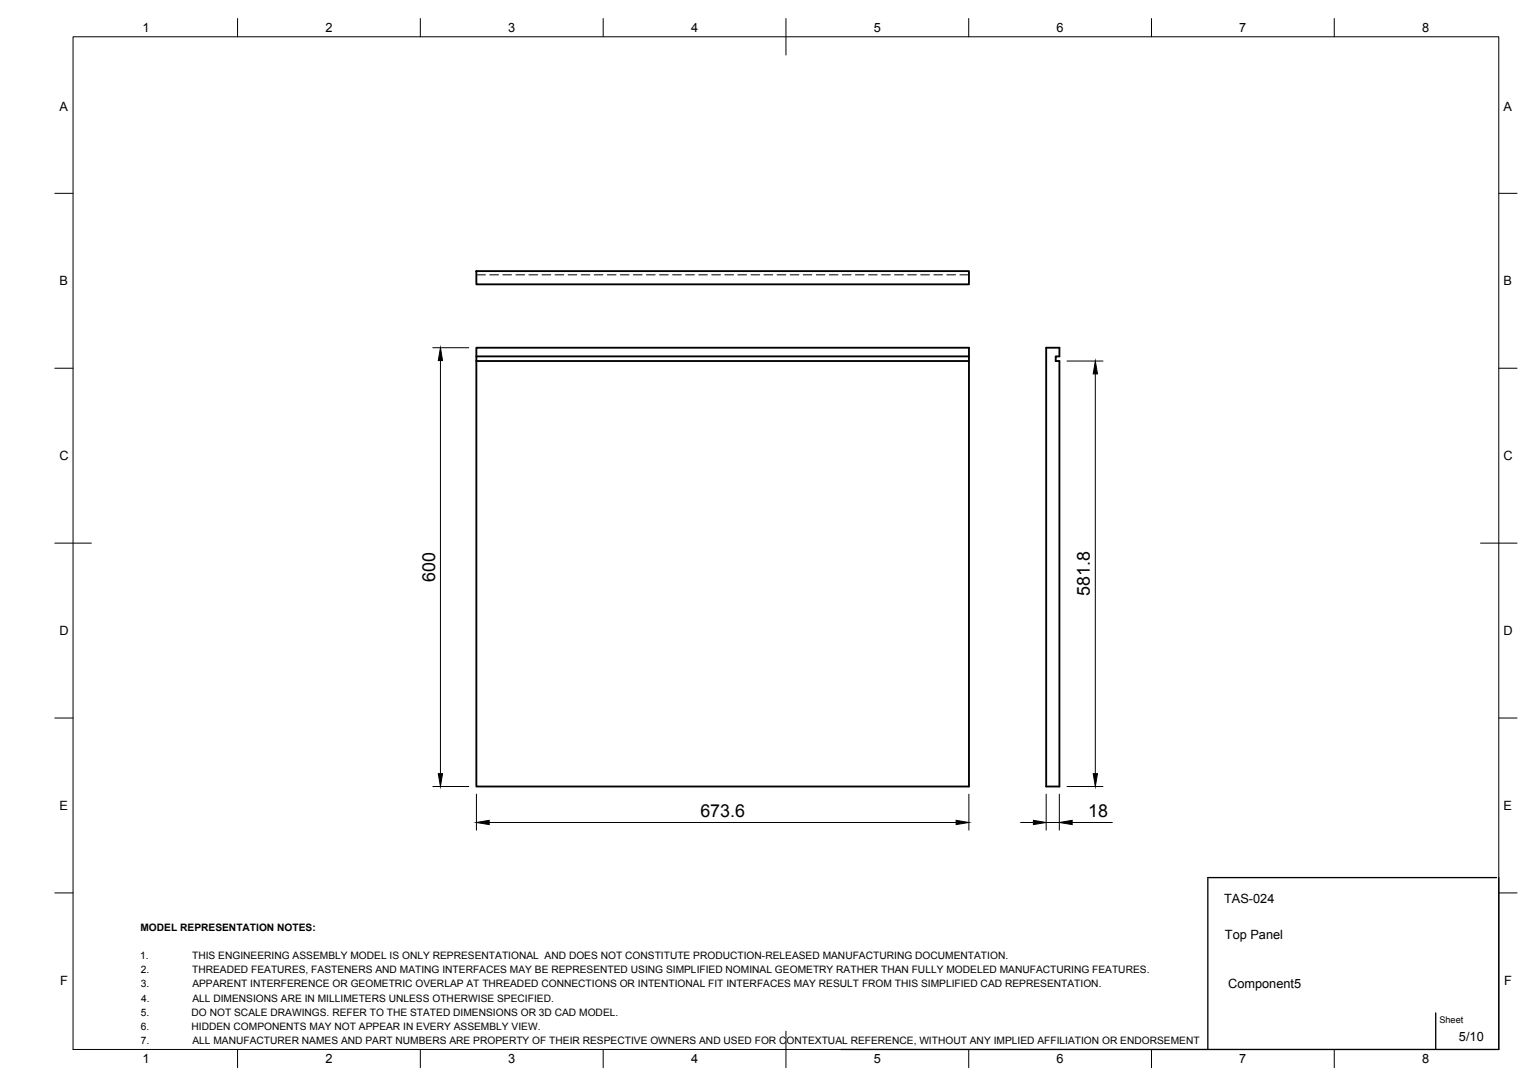
ISO-10303-21;
HEADER;
/* Generated by software containing ST-Developer
 * from STEP Tools, Inc. (www.steptools.com) 
 */

FILE_DESCRIPTION(
/* description */ (''),
/* implementation_level */ '2;1');

FILE_NAME(
/* name */ 'Top panel.step',
/* time_stamp */ '2026-11-15T17:53:25-08:00',
/* author */ (''),
/* organization */ (''),
/* preprocessor_version */ 'ST-DEVELOPER v20.2',
/* originating_system */ 'Autodesk Translation Framework v15.17.0.0',
/* authorisation */ '');

FILE_SCHEMA (('AUTOMOTIVE_DESIGN { 1 0 10303 214 3 1 1 }'));
ENDSEC;

DATA;
#10=MECHANICAL_DESIGN_GEOMETRIC_PRESENTATION_REPRESENTATION('',(#133),#2673);
#117=SHAPE_REPRESENTATION_RELATIONSHIP('SRR','None',#2725,#125);
#125=ADVANCED_BREP_SHAPE_REPRESENTATION('',(#141),#2667);
#133=STYLED_ITEM('',(#2774),#141);
#141=MANIFOLD_SOLID_BREP('Body1',#1519);
#202=PLANE('',#1690);
#203=PLANE('',#1691);
#204=PLANE('',#1692);
#205=PLANE('',#1693);
#206=PLANE('',#1694);
#207=PLANE('',#1695);
#208=PLANE('',#1696);
#209=PLANE('',#1697);
#210=PLANE('',#1698);
#211=PLANE('',#1699);
#285=FACE_OUTER_BOUND('',#384,.T.);
#286=FACE_OUTER_BOUND('',#385,.T.);
#287=FACE_OUTER_BOUND('',#386,.T.);
#288=FACE_OUTER_BOUND('',#387,.T.);
#289=FACE_OUTER_BOUND('',#388,.T.);
#290=FACE_OUTER_BOUND('',#389,.T.);
#291=FACE_OUTER_BOUND('',#390,.T.);
#292=FACE_OUTER_BOUND('',#391,.T.);
#293=FACE_OUTER_BOUND('',#392,.T.);
#294=FACE_OUTER_BOUND('',#393,.T.);
#384=EDGE_LOOP('',(#1280,#1281,#1282,#1283));
#385=EDGE_LOOP('',(#1284,#1285,#1286,#1287));
#386=EDGE_LOOP('',(#1288,#1289,#1290,#1291));
#387=EDGE_LOOP('',(#1292,#1293,#1294,#1295,#1296,#1297,#1298,#1299));
#388=EDGE_LOOP('',(#1300,#1301,#1302,#1303));
#389=EDGE_LOOP('',(#1304,#1305,#1306,#1307));
#390=EDGE_LOOP('',(#1308,#1309,#1310,#1311));
#391=EDGE_LOOP('',(#1312,#1313,#1314,#1315,#1316,#1317,#1318,#1319));
#392=EDGE_LOOP('',(#1320,#1321,#1322,#1323));
#393=EDGE_LOOP('',(#1324,#1325,#1326,#1327));
#518=LINE('',#2479,#666);
#519=LINE('',#2481,#667);
#520=LINE('',#2483,#668);
#521=LINE('',#2484,#669);
#522=LINE('',#2488,#670);
#523=LINE('',#2490,#671);
#524=LINE('',#2492,#672);
#525=LINE('',#2493,#673);
#526=LINE('',#2495,#674);
#527=LINE('',#2496,#675);
#528=LINE('',#2499,#676);
#529=LINE('',#2501,#677);
#530=LINE('',#2503,#678);
#531=LINE('',#2505,#679);
#532=LINE('',#2506,#680);
#533=LINE('',#2509,#681);
#534=LINE('',#2510,#682);
#535=LINE('',#2513,#683);
#536=LINE('',#2515,#684);
#537=LINE('',#2516,#685);
#538=LINE('',#2519,#686);
#539=LINE('',#2520,#687);
#540=LINE('',#2522,#688);
#541=LINE('',#2523,#689);
#666=VECTOR('',#2018,1.);
#667=VECTOR('',#2019,1.);
#668=VECTOR('',#2020,1.);
#669=VECTOR('',#2021,1.);
#670=VECTOR('',#2024,1.);
#671=VECTOR('',#2025,1.);
#672=VECTOR('',#2026,1.);
#673=VECTOR('',#2027,1.);
#674=VECTOR('',#2030,1.);
#675=VECTOR('',#2031,1.);
#676=VECTOR('',#2034,1.);
#677=VECTOR('',#2035,1.);
#678=VECTOR('',#2036,1.);
#679=VECTOR('',#2037,1.);
#680=VECTOR('',#2038,1.);
#681=VECTOR('',#2041,1.);
#682=VECTOR('',#2042,1.);
#683=VECTOR('',#2045,1.);
#684=VECTOR('',#2046,1.);
#685=VECTOR('',#2047,1.);
#686=VECTOR('',#2050,1.);
#687=VECTOR('',#2051,1.);
#688=VECTOR('',#2054,1.);
#689=VECTOR('',#2055,1.);
#828=VERTEX_POINT('',#2477);
#829=VERTEX_POINT('',#2478);
#830=VERTEX_POINT('',#2480);
#831=VERTEX_POINT('',#2482);
#832=VERTEX_POINT('',#2486);
#833=VERTEX_POINT('',#2487);
#834=VERTEX_POINT('',#2489);
#835=VERTEX_POINT('',#2491);
#836=VERTEX_POINT('',#2498);
#837=VERTEX_POINT('',#2500);
#838=VERTEX_POINT('',#2502);
#839=VERTEX_POINT('',#2504);
#840=VERTEX_POINT('',#2508);
#841=VERTEX_POINT('',#2512);
#842=VERTEX_POINT('',#2514);
#843=VERTEX_POINT('',#2518);
#986=EDGE_CURVE('',#828,#829,#518,.T.);
#987=EDGE_CURVE('',#830,#828,#519,.T.);
#988=EDGE_CURVE('',#831,#830,#520,.T.);
#989=EDGE_CURVE('',#829,#831,#521,.T.);
#990=EDGE_CURVE('',#832,#833,#522,.T.);
#991=EDGE_CURVE('',#834,#832,#523,.T.);
#992=EDGE_CURVE('',#835,#834,#524,.T.);
#993=EDGE_CURVE('',#833,#835,#525,.T.);
#994=EDGE_CURVE('',#831,#834,#526,.T.);
#995=EDGE_CURVE('',#835,#830,#527,.T.);
#996=EDGE_CURVE('',#836,#828,#528,.T.);
#997=EDGE_CURVE('',#837,#836,#529,.T.);
#998=EDGE_CURVE('',#837,#838,#530,.T.);
#999=EDGE_CURVE('',#838,#839,#531,.T.);
#1000=EDGE_CURVE('',#833,#839,#532,.T.);
#1001=EDGE_CURVE('',#829,#840,#533,.T.);
#1002=EDGE_CURVE('',#840,#836,#534,.T.);
#1003=EDGE_CURVE('',#838,#841,#535,.T.);
#1004=EDGE_CURVE('',#841,#842,#536,.T.);
#1005=EDGE_CURVE('',#839,#842,#537,.T.);
#1006=EDGE_CURVE('',#843,#837,#538,.T.);
#1007=EDGE_CURVE('',#843,#840,#539,.T.);
#1008=EDGE_CURVE('',#842,#832,#540,.T.);
#1009=EDGE_CURVE('',#841,#843,#541,.T.);
#1280=ORIENTED_EDGE('',*,*,#986,.F.);
#1281=ORIENTED_EDGE('',*,*,#987,.F.);
#1282=ORIENTED_EDGE('',*,*,#988,.F.);
#1283=ORIENTED_EDGE('',*,*,#989,.F.);
#1284=ORIENTED_EDGE('',*,*,#990,.F.);
#1285=ORIENTED_EDGE('',*,*,#991,.F.);
#1286=ORIENTED_EDGE('',*,*,#992,.F.);
#1287=ORIENTED_EDGE('',*,*,#993,.F.);
#1288=ORIENTED_EDGE('',*,*,#994,.F.);
#1289=ORIENTED_EDGE('',*,*,#988,.T.);
#1290=ORIENTED_EDGE('',*,*,#995,.F.);
#1291=ORIENTED_EDGE('',*,*,#992,.T.);
#1292=ORIENTED_EDGE('',*,*,#993,.T.);
#1293=ORIENTED_EDGE('',*,*,#995,.T.);
#1294=ORIENTED_EDGE('',*,*,#987,.T.);
#1295=ORIENTED_EDGE('',*,*,#996,.F.);
#1296=ORIENTED_EDGE('',*,*,#997,.F.);
#1297=ORIENTED_EDGE('',*,*,#998,.T.);
#1298=ORIENTED_EDGE('',*,*,#999,.T.);
#1299=ORIENTED_EDGE('',*,*,#1000,.F.);
#1300=ORIENTED_EDGE('',*,*,#986,.T.);
#1301=ORIENTED_EDGE('',*,*,#1001,.T.);
#1302=ORIENTED_EDGE('',*,*,#1002,.T.);
#1303=ORIENTED_EDGE('',*,*,#996,.T.);
#1304=ORIENTED_EDGE('',*,*,#1003,.T.);
#1305=ORIENTED_EDGE('',*,*,#1004,.T.);
#1306=ORIENTED_EDGE('',*,*,#1005,.F.);
#1307=ORIENTED_EDGE('',*,*,#999,.F.);
#1308=ORIENTED_EDGE('',*,*,#1006,.T.);
#1309=ORIENTED_EDGE('',*,*,#997,.T.);
#1310=ORIENTED_EDGE('',*,*,#1002,.F.);
#1311=ORIENTED_EDGE('',*,*,#1007,.F.);
#1312=ORIENTED_EDGE('',*,*,#991,.T.);
#1313=ORIENTED_EDGE('',*,*,#1008,.F.);
#1314=ORIENTED_EDGE('',*,*,#1004,.F.);
#1315=ORIENTED_EDGE('',*,*,#1009,.T.);
#1316=ORIENTED_EDGE('',*,*,#1007,.T.);
#1317=ORIENTED_EDGE('',*,*,#1001,.F.);
#1318=ORIENTED_EDGE('',*,*,#989,.T.);
#1319=ORIENTED_EDGE('',*,*,#994,.T.);
#1320=ORIENTED_EDGE('',*,*,#990,.T.);
#1321=ORIENTED_EDGE('',*,*,#1000,.T.);
#1322=ORIENTED_EDGE('',*,*,#1005,.T.);
#1323=ORIENTED_EDGE('',*,*,#1008,.T.);
#1324=ORIENTED_EDGE('',*,*,#1009,.F.);
#1325=ORIENTED_EDGE('',*,*,#1003,.F.);
#1326=ORIENTED_EDGE('',*,*,#998,.F.);
#1327=ORIENTED_EDGE('',*,*,#1006,.F.);
#1480=ADVANCED_FACE('',(#285),#202,.F.);
#1481=ADVANCED_FACE('',(#286),#203,.F.);
#1482=ADVANCED_FACE('',(#287),#204,.T.);
#1483=ADVANCED_FACE('',(#288),#205,.T.);
#1484=ADVANCED_FACE('',(#289),#206,.T.);
#1485=ADVANCED_FACE('',(#290),#207,.T.);
#1486=ADVANCED_FACE('',(#291),#208,.T.);
#1487=ADVANCED_FACE('',(#292),#209,.T.);
#1488=ADVANCED_FACE('',(#293),#210,.T.);
#1489=ADVANCED_FACE('',(#294),#211,.F.);
#1519=CLOSED_SHELL('',(#1480,#1481,#1482,#1483,#1484,#1485,#1486,#1487,
#1488,#1489));
#1689=AXIS2_PLACEMENT_3D('',#2475,#2014,#2015);
#1690=AXIS2_PLACEMENT_3D('',#2476,#2016,#2017);
#1691=AXIS2_PLACEMENT_3D('',#2485,#2022,#2023);
#1692=AXIS2_PLACEMENT_3D('',#2494,#2028,#2029);
#1693=AXIS2_PLACEMENT_3D('',#2497,#2032,#2033);
#1694=AXIS2_PLACEMENT_3D('',#2507,#2039,#2040);
#1695=AXIS2_PLACEMENT_3D('',#2511,#2043,#2044);
#1696=AXIS2_PLACEMENT_3D('',#2517,#2048,#2049);
#1697=AXIS2_PLACEMENT_3D('',#2521,#2052,#2053);
#1698=AXIS2_PLACEMENT_3D('',#2524,#2056,#2057);
#1699=AXIS2_PLACEMENT_3D('',#2525,#2058,#2059);
#2014=DIRECTION('axis',(0.,0.,1.));
#2015=DIRECTION('refdir',(1.,0.,0.));
#2016=DIRECTION('center_axis',(0.,-1.,0.));
#2017=DIRECTION('ref_axis',(1.,0.,0.));
#2018=DIRECTION('',(-1.,0.,0.));
#2019=DIRECTION('',(0.,0.,1.));
#2020=DIRECTION('',(1.,0.,0.));
#2021=DIRECTION('',(0.,0.,-1.));
#2022=DIRECTION('center_axis',(0.,1.,0.));
#2023=DIRECTION('ref_axis',(-1.,0.,0.));
#2024=DIRECTION('',(1.,0.,0.));
#2025=DIRECTION('',(0.,0.,1.));
#2026=DIRECTION('',(-1.,0.,0.));
#2027=DIRECTION('',(0.,0.,-1.));
#2028=DIRECTION('center_axis',(0.,0.,1.));
#2029=DIRECTION('ref_axis',(1.,0.,0.));
#2030=DIRECTION('',(0.,1.,0.));
#2031=DIRECTION('',(0.,-1.,0.));
#2032=DIRECTION('center_axis',(1.,0.,0.));
#2033=DIRECTION('ref_axis',(0.,1.,0.));
#2034=DIRECTION('',(0.,1.,0.));
#2035=DIRECTION('',(0.,0.,1.));
#2036=DIRECTION('',(0.,1.,0.));
#2037=DIRECTION('',(0.,0.,1.));
#2038=DIRECTION('',(0.,1.,0.));
#2039=DIRECTION('center_axis',(0.,0.,1.));
#2040=DIRECTION('ref_axis',(1.,0.,0.));
#2041=DIRECTION('',(0.,-1.,0.));
#2042=DIRECTION('',(1.,0.,0.));
#2043=DIRECTION('center_axis',(0.,1.,0.));
#2044=DIRECTION('ref_axis',(-1.,0.,0.));
#2045=DIRECTION('',(-1.,0.,0.));
#2046=DIRECTION('',(0.,0.,1.));
#2047=DIRECTION('',(-1.,0.,0.));
#2048=DIRECTION('center_axis',(0.,-1.,0.));
#2049=DIRECTION('ref_axis',(1.,0.,0.));
#2050=DIRECTION('',(1.,0.,0.));
#2051=DIRECTION('',(0.,0.,1.));
#2052=DIRECTION('center_axis',(-1.,0.,0.));
#2053=DIRECTION('ref_axis',(0.,-1.,0.));
#2054=DIRECTION('',(0.,-1.,0.));
#2055=DIRECTION('',(0.,-1.,0.));
#2056=DIRECTION('center_axis',(0.,0.,1.));
#2057=DIRECTION('ref_axis',(1.,0.,0.));
#2058=DIRECTION('center_axis',(0.,0.,1.));
#2059=DIRECTION('ref_axis',(1.,0.,0.));
#2475=CARTESIAN_POINT('',(0.,0.,0.));
#2476=CARTESIAN_POINT('Origin',(0.,58.18,1.3));
#2477=CARTESIAN_POINT('',(67.36,58.18,1.8));
#2478=CARTESIAN_POINT('',(0.,58.18,1.8));
#2479=CARTESIAN_POINT('',(16.84,58.18,1.8));
#2480=CARTESIAN_POINT('',(67.36,58.18,1.3));
#2481=CARTESIAN_POINT('',(67.36,58.18,0.65));
#2482=CARTESIAN_POINT('',(0.,58.18,1.3));
#2483=CARTESIAN_POINT('',(0.,58.18,1.3));
#2484=CARTESIAN_POINT('',(0.,58.18,0.65));
#2485=CARTESIAN_POINT('Origin',(67.36,58.82,1.3));
#2486=CARTESIAN_POINT('',(0.,58.82,1.8));
#2487=CARTESIAN_POINT('',(67.36,58.82,1.8));
#2488=CARTESIAN_POINT('',(50.52,58.82,1.8));
#2489=CARTESIAN_POINT('',(0.,58.82,1.3));
#2490=CARTESIAN_POINT('',(0.,58.82,0.65));
#2491=CARTESIAN_POINT('',(67.36,58.82,1.3));
#2492=CARTESIAN_POINT('',(67.36,58.82,1.3));
#2493=CARTESIAN_POINT('',(67.36,58.82,0.65));
#2494=CARTESIAN_POINT('Origin',(33.68,58.5,1.3));
#2495=CARTESIAN_POINT('',(0.,59.25,1.3));
#2496=CARTESIAN_POINT('',(67.36,29.25,1.3));
#2497=CARTESIAN_POINT('Origin',(67.36,0.,0.));
#2498=CARTESIAN_POINT('',(67.36,0.,1.8));
#2499=CARTESIAN_POINT('',(67.36,0.,1.8));
#2500=CARTESIAN_POINT('',(67.36,0.,0.));
#2501=CARTESIAN_POINT('',(67.36,0.,0.));
#2502=CARTESIAN_POINT('',(67.36,60.,0.));
#2503=CARTESIAN_POINT('',(67.36,0.,0.));
#2504=CARTESIAN_POINT('',(67.36,60.,1.8));
#2505=CARTESIAN_POINT('',(67.36,60.,0.));
#2506=CARTESIAN_POINT('',(67.36,0.,1.8));
#2507=CARTESIAN_POINT('Origin',(33.68,30.,1.8));
#2508=CARTESIAN_POINT('',(0.,0.,1.8));
#2509=CARTESIAN_POINT('',(0.,60.,1.8));
#2510=CARTESIAN_POINT('',(0.,0.,1.8));
#2511=CARTESIAN_POINT('Origin',(67.36,60.,0.));
#2512=CARTESIAN_POINT('',(0.,60.,0.));
#2513=CARTESIAN_POINT('',(67.36,60.,0.));
#2514=CARTESIAN_POINT('',(0.,60.,1.8));
#2515=CARTESIAN_POINT('',(0.,60.,0.));
#2516=CARTESIAN_POINT('',(67.36,60.,1.8));
#2517=CARTESIAN_POINT('Origin',(0.,0.,0.));
#2518=CARTESIAN_POINT('',(0.,0.,0.));
#2519=CARTESIAN_POINT('',(0.,0.,0.));
#2520=CARTESIAN_POINT('',(0.,0.,0.));
#2521=CARTESIAN_POINT('Origin',(0.,60.,0.));
#2522=CARTESIAN_POINT('',(0.,60.,1.8));
#2523=CARTESIAN_POINT('',(0.,60.,0.));
#2524=CARTESIAN_POINT('Origin',(33.68,30.,1.8));
#2525=CARTESIAN_POINT('Origin',(33.68,30.,0.));
#2657=UNCERTAINTY_MEASURE_WITH_UNIT(LENGTH_MEASURE(0.001),#2674,
'DISTANCE_ACCURACY_VALUE',
'Maximum model space distance between geometric entities at asserted c
onnectivities');
#2663=UNCERTAINTY_MEASURE_WITH_UNIT(LENGTH_MEASURE(0.001),#2674,
'DISTANCE_ACCURACY_VALUE',
'Maximum model space distance between geometric entities at asserted c
onnectivities');
#2667=(
GEOMETRIC_REPRESENTATION_CONTEXT(3)
GLOBAL_UNCERTAINTY_ASSIGNED_CONTEXT((#2657))
GLOBAL_UNIT_ASSIGNED_CONTEXT((#2674,#2676,#2677))
REPRESENTATION_CONTEXT('','3D')
);
#2673=(
GEOMETRIC_REPRESENTATION_CONTEXT(3)
GLOBAL_UNCERTAINTY_ASSIGNED_CONTEXT((#2663))
GLOBAL_UNIT_ASSIGNED_CONTEXT((#2674,#2676,#2677))
REPRESENTATION_CONTEXT('','3D')
);
#2674=(
LENGTH_UNIT()
NAMED_UNIT(*)
SI_UNIT(.CENTI.,.METRE.)
);
#2676=(
NAMED_UNIT(*)
PLANE_ANGLE_UNIT()
SI_UNIT($,.RADIAN.)
);
#2677=(
NAMED_UNIT(*)
SI_UNIT($,.STERADIAN.)
SOLID_ANGLE_UNIT()
);
#2681=SHAPE_DEFINITION_REPRESENTATION(#2690,#2725);
#2690=PRODUCT_DEFINITION_SHAPE('',$,#2735);
#2725=SHAPE_REPRESENTATION('',(#1689),#2667);
#2731=PRODUCT_DEFINITION_CONTEXT('part definition',#2760,'design');
#2735=PRODUCT_DEFINITION('Top Panel','Top panel',#2744,#2731);
#2744=PRODUCT_DEFINITION_FORMATION('',$,#2765);
#2760=APPLICATION_CONTEXT(
'Core Data for Automotive Mechanical Design Process');
#2761=PRODUCT_CONTEXT('part definition',#2760,'mechanical');
#2765=PRODUCT('Top Panel','Top panel',$,(#2761));
#2774=PRESENTATION_STYLE_ASSIGNMENT((#2783));
#2783=SURFACE_STYLE_USAGE(.BOTH.,#2792);
#2792=SURFACE_SIDE_STYLE('',(#2801));
#2801=SURFACE_STYLE_FILL_AREA(#2810);
#2810=FILL_AREA_STYLE('Top panel finish',(#2819));
#2819=FILL_AREA_STYLE_COLOUR('Top panel finish',#2828);
#2828=COLOUR_RGB('Top panel finish',0.662745098039216,0.823529411764706,
0.917647058823529);
ENDSEC;
END-ISO-10303-21;
